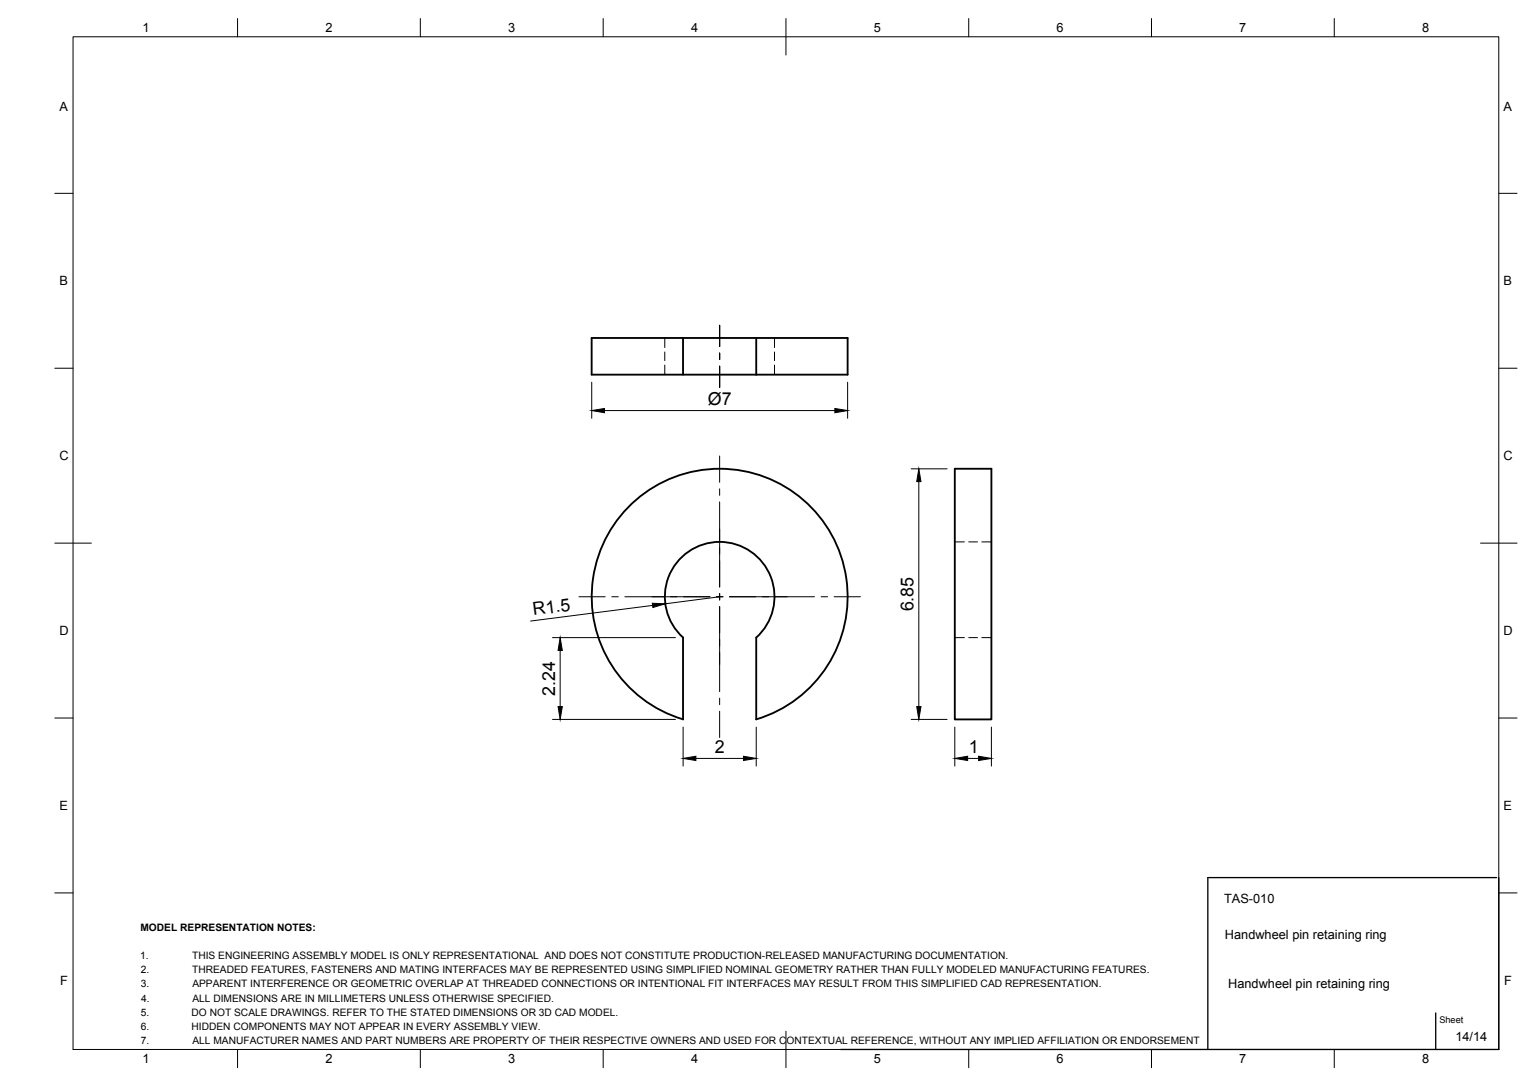
ISO-10303-21;
HEADER;
/* Generated by software containing ST-Developer
 * from STEP Tools, Inc. (www.steptools.com) 
 */

FILE_DESCRIPTION(
/* description */ (
'Independent keyed-quill tailstock, native coupled50mm slider andM16x2
 feed screw, conical dead center, bronze sleeves/thrust washers, cross
-pinned handwheel and bolted guide key. Custom center taper; no standa
rd taper compatibility, machine-bed compatibility or load rating assig
ned.'),
/* implementation_level */ '2;1');

FILE_NAME(
/* name */ 'Handwheel pin retaining ring.step',
/* time_stamp */ '2026-11-14T07:17:36-08:00',
/* author */ (''),
/* organization */ (''),
/* preprocessor_version */ 'ST-DEVELOPER v20.2',
/* originating_system */ 'Autodesk Translation Framework v15.17.0.0',
/* authorisation */ '');

FILE_SCHEMA (('AUTOMOTIVE_DESIGN { 1 0 10303 214 3 1 1 }'));
ENDSEC;

DATA;
#10=MECHANICAL_DESIGN_GEOMETRIC_PRESENTATION_REPRESENTATION('',(#165),#289387);
#131=SHAPE_REPRESENTATION_RELATIONSHIP('SRR','None',#289466,#148);
#148=ADVANCED_BREP_SHAPE_REPRESENTATION('',(#182),#289382);
#165=STYLED_ITEM('',(#289553),#182);
#182=MANIFOLD_SOLID_BREP('Body1',#16853);
#387=PLANE('',#17728);
#388=PLANE('',#17729);
#389=PLANE('',#17730);
#390=PLANE('',#17737);
#969=FACE_OUTER_BOUND('',#1697,.T.);
#970=FACE_OUTER_BOUND('',#1698,.T.);
#971=FACE_OUTER_BOUND('',#1699,.T.);
#972=FACE_OUTER_BOUND('',#1700,.T.);
#973=FACE_OUTER_BOUND('',#1701,.T.);
#974=FACE_OUTER_BOUND('',#1702,.T.);
#1697=EDGE_LOOP('',(#14809,#14810,#14811,#14812));
#1698=EDGE_LOOP('',(#14813,#14814,#14815,#14816));
#1699=EDGE_LOOP('',(#14817,#14818,#14819,#14820));
#1700=EDGE_LOOP('',(#14821,#14822,#14823,#14824));
#1701=EDGE_LOOP('',(#14825,#14826,#14827,#14828));
#1702=EDGE_LOOP('',(#14829,#14830,#14831,#14832));
#1955=CIRCLE('',#17731,3.5);
#1956=CIRCLE('',#17732,1.5);
#1957=CIRCLE('',#17734,1.5);
#1958=CIRCLE('',#17736,3.5);
#4462=LINE('',#247310,#5099);
#4463=LINE('',#247312,#5100);
#4464=LINE('',#247314,#5101);
#4465=LINE('',#247315,#5102);
#4466=LINE('',#247319,#5103);
#4467=LINE('',#247321,#5104);
#4468=LINE('',#247323,#5105);
#4469=LINE('',#247324,#5106);
#5099=VECTOR('',#19776,10.);
#5100=VECTOR('',#19777,10.);
#5101=VECTOR('',#19778,10.);
#5102=VECTOR('',#19779,10.);
#5103=VECTOR('',#19782,10.);
#5104=VECTOR('',#19783,10.);
#5105=VECTOR('',#19784,10.);
#5106=VECTOR('',#19785,10.);
#7035=VERTEX_POINT('',#247308);
#7036=VERTEX_POINT('',#247309);
#7037=VERTEX_POINT('',#247311);
#7038=VERTEX_POINT('',#247313);
#7039=VERTEX_POINT('',#247317);
#7040=VERTEX_POINT('',#247318);
#7041=VERTEX_POINT('',#247320);
#7042=VERTEX_POINT('',#247322);
#9716=EDGE_CURVE('',#7035,#7036,#4462,.T.);
#9717=EDGE_CURVE('',#7037,#7035,#4463,.T.);
#9718=EDGE_CURVE('',#7038,#7037,#4464,.T.);
#9719=EDGE_CURVE('',#7036,#7038,#4465,.T.);
#9720=EDGE_CURVE('',#7039,#7040,#4466,.T.);
#9721=EDGE_CURVE('',#7041,#7039,#4467,.T.);
#9722=EDGE_CURVE('',#7042,#7041,#4468,.T.);
#9723=EDGE_CURVE('',#7040,#7042,#4469,.T.);
#9724=EDGE_CURVE('',#7037,#7042,#1955,.T.);
#9725=EDGE_CURVE('',#7040,#7035,#1956,.T.);
#9726=EDGE_CURVE('',#7039,#7036,#1957,.T.);
#9727=EDGE_CURVE('',#7038,#7041,#1958,.T.);
#14809=ORIENTED_EDGE('',*,*,#9716,.F.);
#14810=ORIENTED_EDGE('',*,*,#9717,.F.);
#14811=ORIENTED_EDGE('',*,*,#9718,.F.);
#14812=ORIENTED_EDGE('',*,*,#9719,.F.);
#14813=ORIENTED_EDGE('',*,*,#9720,.F.);
#14814=ORIENTED_EDGE('',*,*,#9721,.F.);
#14815=ORIENTED_EDGE('',*,*,#9722,.F.);
#14816=ORIENTED_EDGE('',*,*,#9723,.F.);
#14817=ORIENTED_EDGE('',*,*,#9723,.T.);
#14818=ORIENTED_EDGE('',*,*,#9724,.F.);
#14819=ORIENTED_EDGE('',*,*,#9717,.T.);
#14820=ORIENTED_EDGE('',*,*,#9725,.F.);
#14821=ORIENTED_EDGE('',*,*,#9720,.T.);
#14822=ORIENTED_EDGE('',*,*,#9725,.T.);
#14823=ORIENTED_EDGE('',*,*,#9716,.T.);
#14824=ORIENTED_EDGE('',*,*,#9726,.F.);
#14825=ORIENTED_EDGE('',*,*,#9722,.T.);
#14826=ORIENTED_EDGE('',*,*,#9727,.F.);
#14827=ORIENTED_EDGE('',*,*,#9718,.T.);
#14828=ORIENTED_EDGE('',*,*,#9724,.T.);
#14829=ORIENTED_EDGE('',*,*,#9721,.T.);
#14830=ORIENTED_EDGE('',*,*,#9726,.T.);
#14831=ORIENTED_EDGE('',*,*,#9719,.T.);
#14832=ORIENTED_EDGE('',*,*,#9727,.T.);
#16134=CYLINDRICAL_SURFACE('',#17733,1.5);
#16135=CYLINDRICAL_SURFACE('',#17735,3.5);
#16737=ADVANCED_FACE('',(#969),#387,.F.);
#16738=ADVANCED_FACE('',(#970),#388,.F.);
#16739=ADVANCED_FACE('',(#971),#389,.F.);
#16740=ADVANCED_FACE('',(#972),#16134,.F.);
#16741=ADVANCED_FACE('',(#973),#16135,.T.);
#16742=ADVANCED_FACE('',(#974),#390,.T.);
#16853=CLOSED_SHELL('',(#16737,#16738,#16739,#16740,#16741,#16742));
#17727=AXIS2_PLACEMENT_3D('',#247306,#19772,#19773);
#17728=AXIS2_PLACEMENT_3D('',#247307,#19774,#19775);
#17729=AXIS2_PLACEMENT_3D('',#247316,#19780,#19781);
#17730=AXIS2_PLACEMENT_3D('',#247325,#19786,#19787);
#17731=AXIS2_PLACEMENT_3D('',#247326,#19788,#19789);
#17732=AXIS2_PLACEMENT_3D('',#247327,#19790,#19791);
#17733=AXIS2_PLACEMENT_3D('',#247328,#19792,#19793);
#17734=AXIS2_PLACEMENT_3D('',#247329,#19794,#19795);
#17735=AXIS2_PLACEMENT_3D('',#247330,#19796,#19797);
#17736=AXIS2_PLACEMENT_3D('',#247331,#19798,#19799);
#17737=AXIS2_PLACEMENT_3D('',#247332,#19800,#19801);
#19772=DIRECTION('axis',(0.,0.,1.));
#19773=DIRECTION('refdir',(1.,0.,0.));
#19774=DIRECTION('center_axis',(-1.,0.,0.));
#19775=DIRECTION('ref_axis',(0.,1.,0.));
#19776=DIRECTION('',(0.,0.,1.));
#19777=DIRECTION('',(0.,-1.,0.));
#19778=DIRECTION('',(0.,0.,-1.));
#19779=DIRECTION('',(0.,1.,0.));
#19780=DIRECTION('center_axis',(1.,0.,0.));
#19781=DIRECTION('ref_axis',(0.,-1.,0.));
#19782=DIRECTION('',(0.,0.,-1.));
#19783=DIRECTION('',(0.,-1.,0.));
#19784=DIRECTION('',(0.,0.,1.));
#19785=DIRECTION('',(0.,1.,0.));
#19786=DIRECTION('center_axis',(0.,0.,1.));
#19787=DIRECTION('ref_axis',(1.,0.,0.));
#19788=DIRECTION('center_axis',(0.,0.,1.));
#19789=DIRECTION('ref_axis',(1.,0.,0.));
#19790=DIRECTION('center_axis',(0.,0.,-1.));
#19791=DIRECTION('ref_axis',(1.,0.,0.));
#19792=DIRECTION('center_axis',(0.,0.,1.));
#19793=DIRECTION('ref_axis',(6.12323399573677E-17,-1.,0.));
#19794=DIRECTION('center_axis',(0.,0.,-1.));
#19795=DIRECTION('ref_axis',(1.,0.,0.));
#19796=DIRECTION('center_axis',(0.,0.,1.));
#19797=DIRECTION('ref_axis',(6.12323399573677E-17,-1.,0.));
#19798=DIRECTION('center_axis',(0.,0.,1.));
#19799=DIRECTION('ref_axis',(1.,0.,0.));
#19800=DIRECTION('center_axis',(0.,0.,1.));
#19801=DIRECTION('ref_axis',(1.,0.,0.));
#247306=CARTESIAN_POINT('',(0.,0.,0.));
#247307=CARTESIAN_POINT('Origin',(-1.,0.,1.));
#247308=CARTESIAN_POINT('',(-1.,1.11803398874989,0.));
#247309=CARTESIAN_POINT('',(-1.,1.11803398874989,1.));
#247310=CARTESIAN_POINT('',(-1.,1.11803398874989,0.));
#247311=CARTESIAN_POINT('',(-1.,3.35410196624968,0.));
#247312=CARTESIAN_POINT('',(-1.,0.,0.));
#247313=CARTESIAN_POINT('',(-1.,3.35410196624968,1.));
#247314=CARTESIAN_POINT('',(-1.,3.35410196624968,0.));
#247315=CARTESIAN_POINT('',(-1.,0.,1.));
#247316=CARTESIAN_POINT('Origin',(1.,7.,1.));
#247317=CARTESIAN_POINT('',(1.,1.11803398874989,1.));
#247318=CARTESIAN_POINT('',(1.,1.11803398874989,0.));
#247319=CARTESIAN_POINT('',(1.,1.11803398874989,0.));
#247320=CARTESIAN_POINT('',(1.,3.35410196624968,1.));
#247321=CARTESIAN_POINT('',(1.,3.5,1.));
#247322=CARTESIAN_POINT('',(1.,3.35410196624968,0.));
#247323=CARTESIAN_POINT('',(1.,3.35410196624968,0.));
#247324=CARTESIAN_POINT('',(1.,3.5,0.));
#247325=CARTESIAN_POINT('Origin',(0.,0.,0.));
#247326=CARTESIAN_POINT('Origin',(0.,0.,0.));
#247327=CARTESIAN_POINT('Origin',(0.,0.,0.));
#247328=CARTESIAN_POINT('Origin',(0.,0.,0.));
#247329=CARTESIAN_POINT('Origin',(0.,0.,1.));
#247330=CARTESIAN_POINT('Origin',(0.,0.,0.));
#247331=CARTESIAN_POINT('Origin',(0.,0.,1.));
#247332=CARTESIAN_POINT('Origin',(0.,0.,1.));
#289363=UNCERTAINTY_MEASURE_WITH_UNIT(LENGTH_MEASURE(0.01),#289388,
'DISTANCE_ACCURACY_VALUE',
'Maximum model space distance between geometric entities at asserted c
onnectivities');
#289368=UNCERTAINTY_MEASURE_WITH_UNIT(LENGTH_MEASURE(0.01),#289388,
'DISTANCE_ACCURACY_VALUE',
'Maximum model space distance between geometric entities at asserted c
onnectivities');
#289382=(
GEOMETRIC_REPRESENTATION_CONTEXT(3)
GLOBAL_UNCERTAINTY_ASSIGNED_CONTEXT((#289363))
GLOBAL_UNIT_ASSIGNED_CONTEXT((#289388,#289390,#289391))
REPRESENTATION_CONTEXT('','3D')
);
#289387=(
GEOMETRIC_REPRESENTATION_CONTEXT(3)
GLOBAL_UNCERTAINTY_ASSIGNED_CONTEXT((#289368))
GLOBAL_UNIT_ASSIGNED_CONTEXT((#289388,#289390,#289391))
REPRESENTATION_CONTEXT('','3D')
);
#289388=(
LENGTH_UNIT()
NAMED_UNIT(*)
SI_UNIT(.MILLI.,.METRE.)
);
#289390=(
NAMED_UNIT(*)
PLANE_ANGLE_UNIT()
SI_UNIT($,.RADIAN.)
);
#289391=(
NAMED_UNIT(*)
SI_UNIT($,.STERADIAN.)
SOLID_ANGLE_UNIT()
);
#289405=SHAPE_DEFINITION_REPRESENTATION(#289423,#289466);
#289423=PRODUCT_DEFINITION_SHAPE('',$,#289485);
#289466=SHAPE_REPRESENTATION('',(#17727),#289382);
#289471=PRODUCT_DEFINITION_CONTEXT('part definition',#289527,'design');
#289485=PRODUCT_DEFINITION('Handwheel pin retaining ring',
'Handwheel pin retaining ring',#289503,#289471);
#289503=PRODUCT_DEFINITION_FORMATION('',$,#289542);
#289527=APPLICATION_CONTEXT(
'Core Data for Automotive Mechanical Design Process');
#289528=PRODUCT_CONTEXT('part definition',#289527,'mechanical');
#289542=PRODUCT('Handwheel pin retaining ring',
'Handwheel pin retaining ring',$,(#289528));
#289553=PRESENTATION_STYLE_ASSIGNMENT((#289560));
#289560=SURFACE_STYLE_USAGE(.BOTH.,#289567);
#289567=SURFACE_SIDE_STYLE('',(#289574));
#289574=SURFACE_STYLE_FILL_AREA(#289581);
#289581=FILL_AREA_STYLE('Opaque(64,72,82)',(#289588));
#289588=FILL_AREA_STYLE_COLOUR('Opaque(64,72,82)',#289595);
#289595=COLOUR_RGB('Opaque(64,72,82)',0.250980392156863,0.282352941176471,
0.32156862745098);
ENDSEC;
END-ISO-10303-21;
